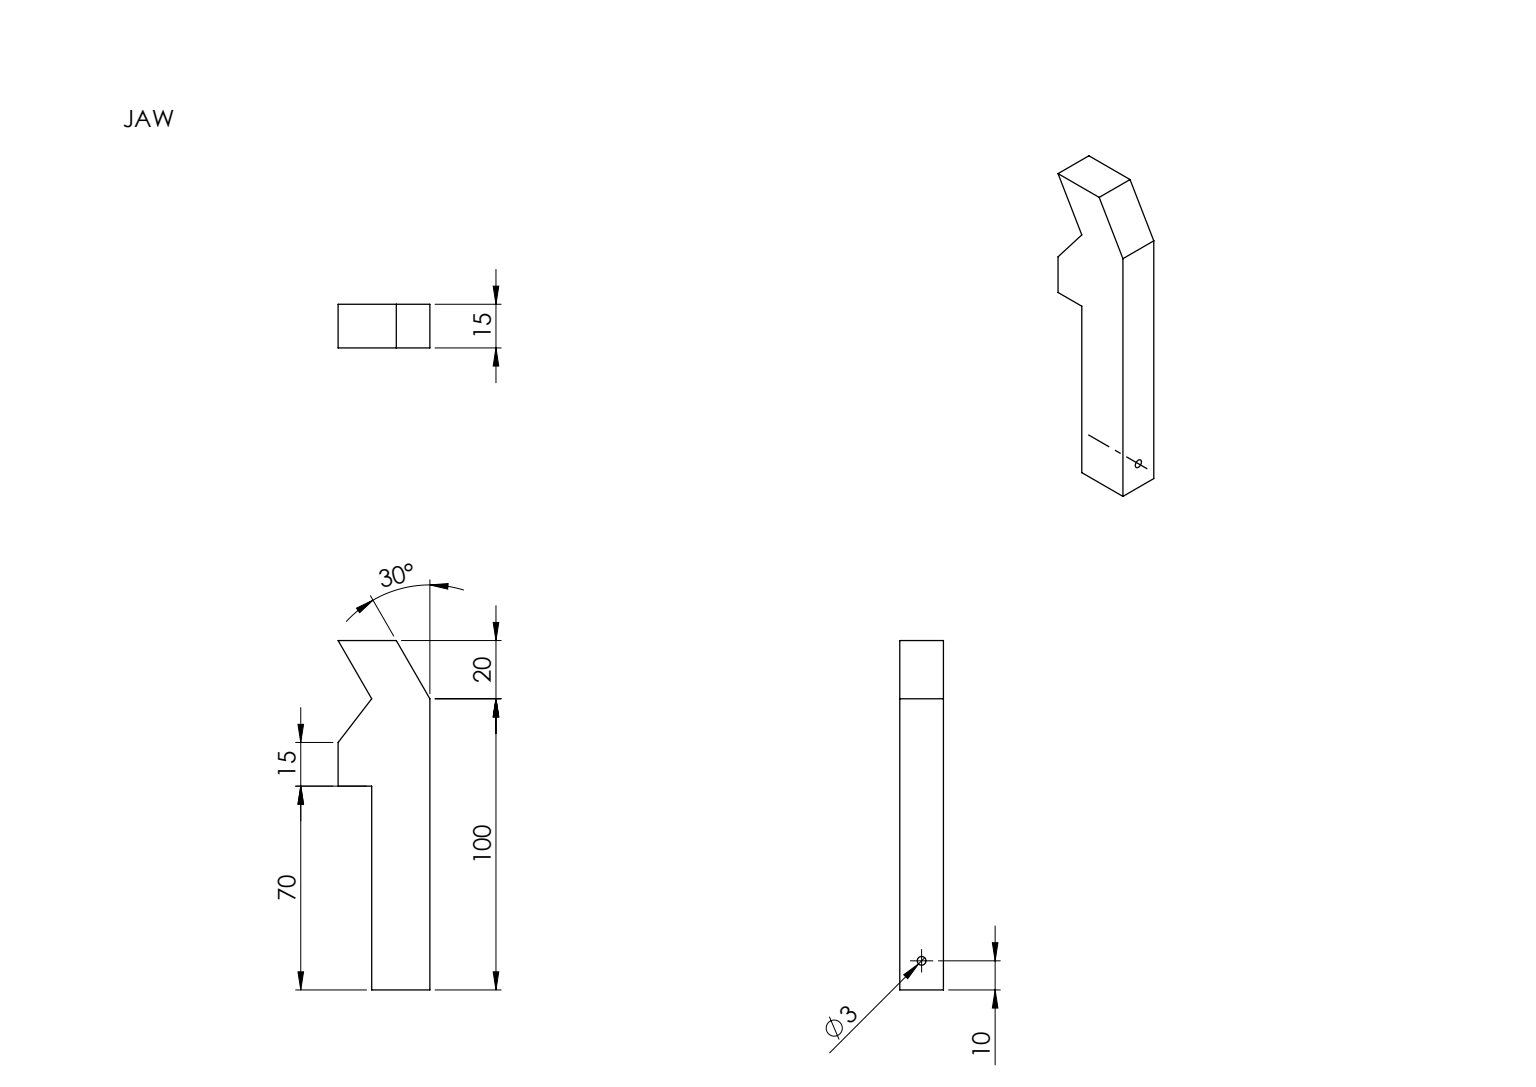
ISO-10303-21;
HEADER;
FILE_DESCRIPTION (('STEP AP214'),
    '1' );
FILE_NAME ('jaw.step',
    '2026-10-04T07:56:41',
    ( '' ),
    ( '' ),
    'SwSTEP 2.0',
    'SolidWorks 2026',
    '' );
FILE_SCHEMA (( 'AUTOMOTIVE_DESIGN' ));
ENDSEC;

DATA;
#13=SHAPE_DEFINITION_REPRESENTATION ( #5408, #1019 ) ;
#38=DIRECTION ( 'NONE',  ( -0.000000000000000000, -0.000000000000000000, -1.000000000000000000 ) ) ;
#42=VECTOR ( 'NONE', #3900, 1000.000000000000000 ) ;
#126=VECTOR ( 'NONE', #38, 1000.000000000000000 ) ;
#181=ORIENTED_EDGE ( 'NONE', *, *, #5142, .F. ) ;
#190=VECTOR ( 'NONE', #1369, 1000.000000000000000 ) ;
#227=ORIENTED_EDGE ( 'NONE', *, *, #6640, .F. ) ;
#250=VERTEX_POINT ( 'NONE', #3258 ) ;
#293=VERTEX_POINT ( 'NONE', #7045 ) ;
#304=ORIENTED_EDGE ( 'NONE', *, *, #4864, .F. ) ;
#353=EDGE_CURVE ( 'NONE', #6629, #3744, #7681, .T. ) ;
#393=CARTESIAN_POINT ( 'NONE',  ( 43.45299461620743386, -9.999999999999994671, 0.000000000000000000 ) ) ;
#417=VERTEX_POINT ( 'NONE', #8308 ) ;
#456=LINE ( 'NONE', #3663, #5763 ) ;
#466=PLANE ( 'NONE',  #7665 ) ;
#515=CIRCLE ( 'NONE', #4553, 1.500000000000000666 ) ;
#524=VERTEX_POINT ( 'NONE', #5948 ) ;
#534=VECTOR ( 'NONE', #7295, 1000.000000000000000 ) ;
#538=CARTESIAN_POINT ( 'NONE',  ( 43.45299461620744097, 100.0000000000000000, -7.500000000000000000 ) ) ;
#539=DIRECTION ( 'NONE',  ( -1.000000000000000000, 0.000000000000000000, 0.000000000000000000 ) ) ;
#549=VERTEX_POINT ( 'NONE', #4695 ) ;
#566=FACE_BOUND ( 'NONE', #6041, .T. ) ;
#573=CARTESIAN_POINT ( 'NONE',  ( 75.00000000000000000, -9.999999999999994671, 1.500000000000000666 ) ) ;
#576=EDGE_CURVE ( 'NONE', #1381, #2388, #1975, .T. ) ;
#579=CARTESIAN_POINT ( 'NONE',  ( 75.00000000000000000, -20.00000000000000000, -7.500000000000000000 ) ) ;
#605=CARTESIAN_POINT ( 'NONE',  ( 43.45299461620743386, 65.00000000000000000, 7.500000000000000000 ) ) ;
#617=ORIENTED_EDGE ( 'NONE', *, *, #2035, .T. ) ;
#635=ADVANCED_FACE ( 'NONE', ( #7236 ), #3406, .F. ) ;
#640=( NAMED_UNIT ( * ) PLANE_ANGLE_UNIT ( ) SI_UNIT ( $, .RADIAN. ) );
#646=VECTOR ( 'NONE', #7811, 1000.000000000000000 ) ;
#649=VECTOR ( 'NONE', #4755, 1000.000000000000000 ) ;
#653=CARTESIAN_POINT ( 'NONE',  ( 43.45299461620743386, 65.00000000000000000, 7.500000000000000000 ) ) ;
#701=ORIENTED_EDGE ( 'NONE', *, *, #4023, .T. ) ;
#712=APPLICATION_CONTEXT ( 'automotive_design' ) ;
#713=DIRECTION ( 'NONE',  ( -0.000000000000000000, -0.000000000000000000, -1.000000000000000000 ) ) ;
#714=LINE ( 'NONE', #5810, #3097 ) ;
#730=SURFACE_STYLE_USAGE ( .BOTH. , #5196 ) ;
#735=DIRECTION ( 'NONE',  ( -0.000000000000000000, 0.000000000000000000, -1.000000000000000000 ) ) ;
#746=ORIENTED_EDGE ( 'NONE', *, *, #4954, .T. ) ;
#773=EDGE_LOOP ( 'NONE', ( #701, #3537, #1533, #746 ) ) ;
#833=CARTESIAN_POINT ( 'NONE',  ( 54.99999999999999289, 80.00000000000000000, -7.500000000000000000 ) ) ;
#880=ORIENTED_EDGE ( 'NONE', *, *, #6640, .T. ) ;
#883=APPLICATION_CONTEXT ( 'automotive_design' ) ;
#896=UNCERTAINTY_MEASURE_WITH_UNIT (LENGTH_MEASURE( 1.000000000000000082E-05 ), #4515, 'distance_accuracy_value', 'NONE');
#906=PLANE ( 'NONE',  #6654 ) ;
#908=CARTESIAN_POINT ( 'NONE',  ( 75.00000000000000000, 80.00000000000000000, 7.500000000000000000 ) ) ;
#912=DIRECTION ( 'NONE',  ( 0.8660254037844380415, 0.5000000000000011102, -0.000000000000000000 ) ) ;
#939=ORIENTED_EDGE ( 'NONE', *, *, #6746, .T. ) ;
#940=CARTESIAN_POINT ( 'NONE',  ( 54.99999999999999289, 80.00000000000000000, -7.500000000000000000 ) ) ;
#949=MECHANICAL_DESIGN_GEOMETRIC_PRESENTATION_REPRESENTATION('',(#1216),#1896);
#955=SURFACE_SIDE_STYLE ('',( #6681 ) ) ;
#990=DIRECTION ( 'NONE',  ( 0.5000000000000011102, -0.8660254037844380415, 0.000000000000000000 ) ) ;
#997=CARTESIAN_POINT ( 'NONE',  ( 63.45299461620744808, 100.0000000000000000, 7.500000000000000000 ) ) ;
#999=ORIENTED_EDGE ( 'NONE', *, *, #7718, .T. ) ;
#1006=VECTOR ( 'NONE', #1758, 1000.000000000000114 ) ;
#1014=EDGE_LOOP ( 'NONE', ( #7055, #2724, #2403, #4042, #1733, #6191, #4300, #4661, #6588 ) ) ;
#1019=SHAPE_REPRESENTATION ( 'jaw', ( #2840 ), #1628 ) ;
#1038=DIRECTION ( 'NONE',  ( -0.000000000000000000, 0.000000000000000000, 1.000000000000000000 ) ) ;
#1049=MECHANICAL_DESIGN_GEOMETRIC_PRESENTATION_REPRESENTATION('',(#4809),#4356);
#1061=CARTESIAN_POINT ( 'NONE',  ( 75.00000000000000000, 80.00000000000000000, 7.500000000000000000 ) ) ;
#1080=ORIENTED_EDGE ( 'NONE', *, *, #5142, .T. ) ;
#1112=VECTOR ( 'NONE', #3807, 1000.000000000000000 ) ;
#1117=LINE ( 'NONE', #7526, #1006 ) ;
#1216=STYLED_ITEM ( 'NONE', ( #5735 ), #7608 ) ;
#1220=DIRECTION ( 'NONE',  ( 1.000000000000000000, -0.000000000000000000, -0.000000000000000000 ) ) ;
#1221=CARTESIAN_POINT ( 'NONE',  ( 75.00000000000000000, -20.00000000000000000, 7.500000000000000000 ) ) ;
#1242=CARTESIAN_POINT ( 'NONE',  ( 43.45299461620743386, -9.999999999999994671, 1.500000000000000666 ) ) ;
#1298=ORIENTED_EDGE ( 'NONE', *, *, #7183, .T. ) ;
#1326=DIRECTION ( 'NONE',  ( 1.000000000000000000, 0.000000000000000000, -0.000000000000000000 ) ) ;
#1369=DIRECTION ( 'NONE',  ( 1.000000000000000000, -0.000000000000000000, -0.000000000000000000 ) ) ;
#1381=VERTEX_POINT ( 'NONE', #5356 ) ;
#1447=ORIENTED_EDGE ( 'NONE', *, *, #5442, .T. ) ;
#1468=AXIS2_PLACEMENT_3D ( 'NONE', #3072, #1220, #4965 ) ;
#1533=ORIENTED_EDGE ( 'NONE', *, *, #7718, .F. ) ;
#1537=FACE_OUTER_BOUND ( 'NONE', #1693, .T. ) ;
#1546=( NAMED_UNIT ( * ) PLANE_ANGLE_UNIT ( ) SI_UNIT ( $, .RADIAN. ) );
#1548=EDGE_CURVE ( 'NONE', #5519, #1381, #5167, .T. ) ;
#1591=DIRECTION ( 'NONE',  ( -0.6099942813304201072, -0.7924058156930603447, 0.000000000000000000 ) ) ;
#1623=VECTOR ( 'NONE', #1650, 1000.000000000000000 ) ;
#1628=( GEOMETRIC_REPRESENTATION_CONTEXT ( 3 ) GLOBAL_UNCERTAINTY_ASSIGNED_CONTEXT ( ( #4856 ) ) GLOBAL_UNIT_ASSIGNED_CONTEXT ( ( #2005, #6383, #3771 ) ) REPRESENTATION_CONTEXT ( 'NONE', 'WORKASPACE' ) );
#1649=VERTEX_POINT ( 'NONE', #573 ) ;
#1650=DIRECTION ( 'NONE',  ( -1.000000000000000000, 0.000000000000000000, 0.000000000000000000 ) ) ;
#1659=EDGE_CURVE ( 'NONE', #250, #417, #4402, .T. ) ;
#1667=CARTESIAN_POINT ( 'NONE',  ( 43.45299461620744097, 100.0000000000000000, -7.500000000000000000 ) ) ;
#1676=VECTOR ( 'NONE', #7231, 1000.000000000000000 ) ;
#1690=MANIFOLD_SOLID_BREP ( 'Cut-Extrude1', #5315 ) ;
#1691=ORIENTED_EDGE ( 'NONE', *, *, #2448, .T. ) ;
#1693=EDGE_LOOP ( 'NONE', ( #2245, #2702, #999, #617, #3311, #7489, #1691, #2350, #6749 ) ) ;
#1721=ADVANCED_FACE ( 'NONE', ( #4785 ), #5294, .F. ) ;
#1725=EDGE_CURVE ( 'NONE', #1381, #6629, #3483, .T. ) ;
#1733=ORIENTED_EDGE ( 'NONE', *, *, #2960, .F. ) ;
#1756=DIRECTION ( 'NONE',  ( 1.000000000000000000, 0.000000000000000000, 0.000000000000000000 ) ) ;
#1758=DIRECTION ( 'NONE',  ( -0.5000000000000011102, 0.8660254037844380415, 0.000000000000000000 ) ) ;
#1781=EDGE_CURVE ( 'NONE', #293, #5112, #4033, .T. ) ;
#1792=LINE ( 'NONE', #5025, #4464 ) ;
#1841=VERTEX_POINT ( 'NONE', #997 ) ;
#1842=LINE ( 'NONE', #7145, #3688 ) ;
#1856=ORIENTED_EDGE ( 'NONE', *, *, #1548, .F. ) ;
#1885=CARTESIAN_POINT ( 'NONE',  ( 54.99999999999999289, 50.00000000000000000, 7.500000000000000000 ) ) ;
#1895=DIRECTION ( 'NONE',  ( 1.000000000000000000, 0.000000000000000000, 0.000000000000000000 ) ) ;
#1896=( GEOMETRIC_REPRESENTATION_CONTEXT ( 3 ) GLOBAL_UNCERTAINTY_ASSIGNED_CONTEXT ( ( #896 ) ) GLOBAL_UNIT_ASSIGNED_CONTEXT ( ( #4515, #640, #7095 ) ) REPRESENTATION_CONTEXT ( 'NONE', 'WORKASPACE' ) );
#1899=ORIENTED_EDGE ( 'NONE', *, *, #4820, .F. ) ;
#1913=ADVANCED_FACE ( 'NONE', ( #4275 ), #2936, .F. ) ;
#1922=VERTEX_POINT ( 'NONE', #3564 ) ;
#1943=ORIENTED_EDGE ( 'NONE', *, *, #2448, .F. ) ;
#1975=LINE ( 'NONE', #7195, #7322 ) ;
#2005=( LENGTH_UNIT ( ) NAMED_UNIT ( * ) SI_UNIT ( .MILLI., .METRE. ) );
#2017=PRODUCT_DEFINITION ( 'UNKNOWN', '', #4690, #4178 ) ;
#2035=EDGE_CURVE ( 'NONE', #8322, #1841, #1117, .T. ) ;
#2076=DIRECTION ( 'NONE',  ( 0.5000000000000011102, -0.8660254037844380415, 0.000000000000000000 ) ) ;
#2097=DIRECTION ( 'NONE',  ( 0.000000000000000000, 0.000000000000000000, -1.000000000000000000 ) ) ;
#2148=ORIENTED_EDGE ( 'NONE', *, *, #3348, .F. ) ;
#2170=EDGE_LOOP ( 'NONE', ( #5540, #6001, #8319, #4192 ) ) ;
#2178=EDGE_CURVE ( 'NONE', #5519, #3650, #1842, .T. ) ;
#2200=EDGE_LOOP ( 'NONE', ( #1298, #7014, #1856, #8055 ) ) ;
#2213=ORIENTED_EDGE ( 'NONE', *, *, #3070, .T. ) ;
#2221=LINE ( 'NONE', #7269, #6382 ) ;
#2245=ORIENTED_EDGE ( 'NONE', *, *, #2667, .T. ) ;
#2271=CARTESIAN_POINT ( 'NONE',  ( 75.00000000000000000, -20.00000000000000000, 7.500000000000000000 ) ) ;
#2323=ORIENTED_EDGE ( 'NONE', *, *, #2035, .F. ) ;
#2334=EDGE_LOOP ( 'NONE', ( #181, #6990 ) ) ;
#2348=VECTOR ( 'NONE', #5444, 1000.000000000000000 ) ;
#2350=ORIENTED_EDGE ( 'NONE', *, *, #1548, .T. ) ;
#2373=LINE ( 'NONE', #4175, #2348 ) ;
#2388=VERTEX_POINT ( 'NONE', #1885 ) ;
#2393=EDGE_CURVE ( 'NONE', #5386, #1649, #4518, .T. ) ;
#2403=ORIENTED_EDGE ( 'NONE', *, *, #7183, .F. ) ;
#2412=CARTESIAN_POINT ( 'NONE',  ( 54.99999999999999289, -20.00000000000000000, 7.500000000000000000 ) ) ;
#2445=ORIENTED_EDGE ( 'NONE', *, *, #7652, .T. ) ;
#2448=EDGE_CURVE ( 'NONE', #524, #5519, #8279, .T. ) ;
#2453=FACE_OUTER_BOUND ( 'NONE', #3610, .T. ) ;
#2455=CARTESIAN_POINT ( 'NONE',  ( 43.45299461620743386, 65.00000000000000000, -7.500000000000000000 ) ) ;
#2467=ORIENTED_EDGE ( 'NONE', *, *, #7477, .T. ) ;
#2471=ORIENTED_EDGE ( 'NONE', *, *, #6088, .T. ) ;
#2488=CARTESIAN_POINT ( 'NONE',  ( 54.99999999999999289, -20.00000000000000000, 7.500000000000000000 ) ) ;
#2507=FILL_AREA_STYLE ('',( #7013 ) ) ;
#2525=PRODUCT ( 'jaw', 'jaw', '', ( #5784 ) ) ;
#2535=DIRECTION ( 'NONE',  ( -0.8660254037844380415, -0.5000000000000011102, 0.000000000000000000 ) ) ;
#2551=CARTESIAN_POINT ( 'NONE',  ( 54.99999999999999289, 80.00000000000000000, 7.500000000000000000 ) ) ;
#2585=CARTESIAN_POINT ( 'NONE',  ( 63.45299461620744808, 100.0000000000000000, 7.500000000000000000 ) ) ;
#2637=EDGE_CURVE ( 'NONE', #1922, #549, #4649, .T. ) ;
#2667=EDGE_CURVE ( 'NONE', #2388, #4058, #2221, .T. ) ;
#2676=CARTESIAN_POINT ( 'NONE',  ( 43.45299461620743386, 65.00000000000000000, -7.500000000000000000 ) ) ;
#2685=CARTESIAN_POINT ( 'NONE',  ( 54.99999999999999289, -9.999999999999994671, 0.000000000000000000 ) ) ;
#2702=ORIENTED_EDGE ( 'NONE', *, *, #4820, .T. ) ;
#2724=ORIENTED_EDGE ( 'NONE', *, *, #353, .F. ) ;
#2760=ADVANCED_FACE ( 'NONE', ( #1537 ), #906, .T. ) ;
#2783=EDGE_LOOP ( 'NONE', ( #227, #3912, #3895, #4312 ) ) ;
#2801=ORIENTED_EDGE ( 'NONE', *, *, #576, .F. ) ;
#2805=VECTOR ( 'NONE', #3237, 1000.000000000000000 ) ;
#2818=CARTESIAN_POINT ( 'NONE',  ( 63.45299461620744808, 100.0000000000000000, 7.500000000000000000 ) ) ;
#2840=AXIS2_PLACEMENT_3D ( 'NONE', #8120, #5497, #1756 ) ;
#2850=CARTESIAN_POINT ( 'NONE',  ( 0.000000000000000000, 0.000000000000000000, 7.500000000000000000 ) ) ;
#2856=ADVANCED_FACE ( 'NONE', ( #4986 ), #5457, .F. ) ;
#2871=CARTESIAN_POINT ( 'NONE',  ( 75.00000000000000000, -9.999999999999994671, 0.000000000000000000 ) ) ;
#2888=VECTOR ( 'NONE', #7689, 1000.000000000000114 ) ;
#2923=DIRECTION ( 'NONE',  ( 1.000000000000000000, 0.000000000000000000, 0.000000000000000000 ) ) ;
#2936=PLANE ( 'NONE',  #3559 ) ;
#2960=EDGE_CURVE ( 'NONE', #5449, #6860, #4819, .T. ) ;
#3015=VECTOR ( 'NONE', #7593, 1000.000000000000000 ) ;
#3016=UNCERTAINTY_MEASURE_WITH_UNIT (LENGTH_MEASURE( 1.000000000000000082E-05 ), #7238, 'distance_accuracy_value', 'NONE');
#3070=EDGE_CURVE ( 'NONE', #8322, #293, #5574, .T. ) ;
#3072=CARTESIAN_POINT ( 'NONE',  ( 43.45299461620743386, -9.999999999999994671, 0.000000000000000000 ) ) ;
#3097=VECTOR ( 'NONE', #6576, 1000.000000000000000 ) ;
#3126=EDGE_LOOP ( 'NONE', ( #5435, #6018, #2801, #7528 ) ) ;
#3144=CARTESIAN_POINT ( 'NONE',  ( 54.99999999999999289, 50.00000000000000000, 7.500000000000000000 ) ) ;
#3146=AXIS2_PLACEMENT_3D ( 'NONE', #6708, #7871, #2097 ) ;
#3214=EDGE_CURVE ( 'NONE', #1841, #4787, #5653, .T. ) ;
#3237=DIRECTION ( 'NONE',  ( 9.251858538542971828E-16, -1.000000000000000000, 0.000000000000000000 ) ) ;
#3254=CARTESIAN_POINT ( 'NONE',  ( 43.45299461620744808, 50.00000000000000000, 7.500000000000000000 ) ) ;
#3258=CARTESIAN_POINT ( 'NONE',  ( 54.99999999999999289, -20.00000000000000000, -7.500000000000000000 ) ) ;
#3311=ORIENTED_EDGE ( 'NONE', *, *, #3214, .T. ) ;
#3338=DIRECTION ( 'NONE',  ( 0.000000000000000000, 1.000000000000000000, 0.000000000000000000 ) ) ;
#3348=EDGE_CURVE ( 'NONE', #4787, #524, #1792, .T. ) ;
#3406=PLANE ( 'NONE',  #5741 ) ;
#3423=CARTESIAN_POINT ( 'NONE',  ( 63.45299461620744808, 100.0000000000000000, -7.500000000000000000 ) ) ;
#3462=CARTESIAN_POINT ( 'NONE',  ( 75.00000000000000000, -20.00000000000000000, 7.500000000000000000 ) ) ;
#3482=ORIENTED_EDGE ( 'NONE', *, *, #5442, .F. ) ;
#3483=LINE ( 'NONE', #7197, #5034 ) ;
#3487=DIRECTION ( 'NONE',  ( 0.000000000000000000, -1.000000000000000000, 0.000000000000000000 ) ) ;
#3537=ORIENTED_EDGE ( 'NONE', *, *, #3070, .F. ) ;
#3559=AXIS2_PLACEMENT_3D ( 'NONE', #4949, #1038, #4874 ) ;
#3564=CARTESIAN_POINT ( 'NONE',  ( 54.99999999999999289, -9.999999999999994671, -1.500000000000000666 ) ) ;
#3610=EDGE_LOOP ( 'NONE', ( #7750, #5914, #1899, #939 ) ) ;
#3623=FACE_OUTER_BOUND ( 'NONE', #4276, .T. ) ;
#3650=VERTEX_POINT ( 'NONE', #2676 ) ;
#3663=CARTESIAN_POINT ( 'NONE',  ( 63.45299461620744808, 100.0000000000000000, 7.500000000000000000 ) ) ;
#3675=LINE ( 'NONE', #2455, #3015 ) ;
#3685=CIRCLE ( 'NONE', #4615, 1.500000000000000666 ) ;
#3688=VECTOR ( 'NONE', #5113, 1000.000000000000000 ) ;
#3716=DIRECTION ( 'NONE',  ( 0.000000000000000000, -0.000000000000000000, 1.000000000000000000 ) ) ;
#3744=VERTEX_POINT ( 'NONE', #6155 ) ;
#3745=DIRECTION ( 'NONE',  ( -0.000000000000000000, -0.000000000000000000, -1.000000000000000000 ) ) ;
#3746=PLANE ( 'NONE',  #5432 ) ;
#3771=( NAMED_UNIT ( * ) SI_UNIT ( $, .STERADIAN. ) SOLID_ANGLE_UNIT ( ) );
#3807=DIRECTION ( 'NONE',  ( -1.000000000000000000, 0.000000000000000000, 0.000000000000000000 ) ) ;
#3815=VECTOR ( 'NONE', #5130, 1000.000000000000000 ) ;
#3852=EDGE_CURVE ( 'NONE', #3744, #250, #2373, .T. ) ;
#3872=ORIENTED_EDGE ( 'NONE', *, *, #7477, .F. ) ;
#3892=AXIS2_PLACEMENT_3D ( 'NONE', #2818, #3487, #7243 ) ;
#3895=ORIENTED_EDGE ( 'NONE', *, *, #6954, .T. ) ;
#3900=DIRECTION ( 'NONE',  ( -0.000000000000000000, -0.000000000000000000, -1.000000000000000000 ) ) ;
#3912=ORIENTED_EDGE ( 'NONE', *, *, #2393, .T. ) ;
#3938=DIRECTION ( 'NONE',  ( 1.000000000000000000, 0.000000000000000000, 0.000000000000000000 ) ) ;
#3944=CARTESIAN_POINT ( 'NONE',  ( 54.99999999999999289, 80.00000000000000000, 7.500000000000000000 ) ) ;
#3965=VECTOR ( 'NONE', #5376, 1000.000000000000114 ) ;
#3966=CARTESIAN_POINT ( 'NONE',  ( 54.99999999999999289, 80.00000000000000000, 7.500000000000000000 ) ) ;
#4006=CARTESIAN_POINT ( 'NONE',  ( 54.99999999999999289, -20.00000000000000000, 7.500000000000000000 ) ) ;
#4023=EDGE_CURVE ( 'NONE', #417, #293, #6401, .T. ) ;
#4032=DIRECTION ( 'NONE',  ( 1.000000000000000000, 0.000000000000000000, 0.000000000000000000 ) ) ;
#4033=LINE ( 'NONE', #5927, #3965 ) ;
#4042=ORIENTED_EDGE ( 'NONE', *, *, #6088, .F. ) ;
#4058=VERTEX_POINT ( 'NONE', #2488 ) ;
#4108=ADVANCED_FACE ( 'NONE', ( #5006, #6277 ), #3746, .F. ) ;
#4112=EDGE_LOOP ( 'NONE', ( #5128, #304, #2148, #2467 ) ) ;
#4136=VECTOR ( 'NONE', #1895, 1000.000000000000000 ) ;
#4155=AXIS2_PLACEMENT_3D ( 'NONE', #1061, #2535, #2076 ) ;
#4175=CARTESIAN_POINT ( 'NONE',  ( 54.99999999999999289, 50.00000000000000000, -7.500000000000000000 ) ) ;
#4178=PRODUCT_DEFINITION_CONTEXT ( 'detailed design', #712, 'design' ) ;
#4180=CARTESIAN_POINT ( 'NONE',  ( 75.00000000000000000, -9.999999999999994671, 0.000000000000000000 ) ) ;
#4192=ORIENTED_EDGE ( 'NONE', *, *, #4808, .T. ) ;
#4257=PLANE ( 'NONE',  #4155 ) ;
#4275=FACE_OUTER_BOUND ( 'NONE', #1014, .T. ) ;
#4276=EDGE_LOOP ( 'NONE', ( #8174, #6317, #4791, #1080 ) ) ;
#4300=ORIENTED_EDGE ( 'NONE', *, *, #1781, .F. ) ;
#4312=ORIENTED_EDGE ( 'NONE', *, *, #2637, .F. ) ;
#4356=( GEOMETRIC_REPRESENTATION_CONTEXT ( 3 ) GLOBAL_UNCERTAINTY_ASSIGNED_CONTEXT ( ( #3016 ) ) GLOBAL_UNIT_ASSIGNED_CONTEXT ( ( #7238, #1546, #7917 ) ) REPRESENTATION_CONTEXT ( 'NONE', 'WORKASPACE' ) );
#4395=PLANE ( 'NONE',  #7317 ) ;
#4402=LINE ( 'NONE', #6981, #4136 ) ;
#4419=VECTOR ( 'NONE', #713, 1000.000000000000000 ) ;
#4438=PLANE ( 'NONE',  #5968 ) ;
#4464=VECTOR ( 'NONE', #5690, 1000.000000000000114 ) ;
#4499=ADVANCED_FACE ( 'NONE', ( #2453 ), #466, .F. ) ;
#4515=( LENGTH_UNIT ( ) NAMED_UNIT ( * ) SI_UNIT ( .MILLI., .METRE. ) );
#4518=LINE ( 'NONE', #1242, #190 ) ;
#4520=LINE ( 'NONE', #7101, #42 ) ;
#4526=DIRECTION ( 'NONE',  ( 0.6099942813304201072, 0.7924058156930603447, 0.000000000000000000 ) ) ;
#4544=LINE ( 'NONE', #3966, #4419 ) ;
#4553=AXIS2_PLACEMENT_3D ( 'NONE', #2871, #5350, #6780 ) ;
#4567=DIRECTION ( 'NONE',  ( 0.7924058156930603447, -0.6099942813304201072, 0.000000000000000000 ) ) ;
#4615=AXIS2_PLACEMENT_3D ( 'NONE', #2685, #1326, #8323 ) ;
#4643=ORIENTED_EDGE ( 'NONE', *, *, #6814, .T. ) ;
#4649=LINE ( 'NONE', #4687, #1676 ) ;
#4660=ADVANCED_FACE ( 'NONE', ( #8303 ), #4257, .F. ) ;
#4661=ORIENTED_EDGE ( 'NONE', *, *, #4023, .F. ) ;
#4687=CARTESIAN_POINT ( 'NONE',  ( 43.45299461620743386, -9.999999999999994671, -1.500000000000000666 ) ) ;
#4690=PRODUCT_DEFINITION_FORMATION_WITH_SPECIFIED_SOURCE ( 'ANY', '', #2525, .NOT_KNOWN. ) ;
#4695=CARTESIAN_POINT ( 'NONE',  ( 75.00000000000000000, -9.999999999999994671, -1.500000000000000666 ) ) ;
#4697=FILL_AREA_STYLE ('',( #6724 ) ) ;
#4738=SURFACE_STYLE_USAGE ( .BOTH. , #955 ) ;
#4755=DIRECTION ( 'NONE',  ( -0.000000000000000000, -0.000000000000000000, -1.000000000000000000 ) ) ;
#4785=FACE_OUTER_BOUND ( 'NONE', #4112, .T. ) ;
#4786=ADVANCED_FACE ( 'NONE', ( #7806 ), #6491, .F. ) ;
#4787=VERTEX_POINT ( 'NONE', #5767 ) ;
#4791=ORIENTED_EDGE ( 'NONE', *, *, #2637, .T. ) ;
#4808=EDGE_CURVE ( 'NONE', #2388, #3744, #7169, .T. ) ;
#4809=STYLED_ITEM ( 'NONE', ( #7277 ), #1690 ) ;
#4819=LINE ( 'NONE', #1667, #6108 ) ;
#4820=EDGE_CURVE ( 'NONE', #4058, #6070, #5138, .T. ) ;
#4831=VECTOR ( 'NONE', #5098, 1000.000000000000000 ) ;
#4856=UNCERTAINTY_MEASURE_WITH_UNIT (LENGTH_MEASURE( 1.000000000000000082E-05 ), #2005, 'distance_accuracy_value', 'NONE');
#4864=EDGE_CURVE ( 'NONE', #524, #6860, #4544, .T. ) ;
#4874=DIRECTION ( 'NONE',  ( 1.000000000000000000, 0.000000000000000000, 0.000000000000000000 ) ) ;
#4945=CARTESIAN_POINT ( 'NONE',  ( 75.00000000000000000, 80.00000000000000000, 7.500000000000000000 ) ) ;
#4949=CARTESIAN_POINT ( 'NONE',  ( 0.000000000000000000, 0.000000000000000000, -7.500000000000000000 ) ) ;
#4954=EDGE_CURVE ( 'NONE', #6070, #417, #6069, .T. ) ;
#4965=DIRECTION ( 'NONE',  ( 0.000000000000000000, 0.000000000000000000, -1.000000000000000000 ) ) ;
#4986=FACE_OUTER_BOUND ( 'NONE', #2783, .T. ) ;
#5006=FACE_BOUND ( 'NONE', #2334, .T. ) ;
#5025=CARTESIAN_POINT ( 'NONE',  ( 43.45299461620744097, 100.0000000000000000, 7.500000000000000000 ) ) ;
#5034=VECTOR ( 'NONE', #6010, 1000.000000000000000 ) ;
#5048=CARTESIAN_POINT ( 'NONE',  ( 54.99999999999999289, -9.999999999999994671, 1.500000000000000666 ) ) ;
#5069=SHAPE_REPRESENTATION_RELATIONSHIP ( 'NONE' , 'NONE' ,  #1019, #7608 ) ;
#5098=DIRECTION ( 'NONE',  ( 1.000000000000000000, 0.000000000000000000, 0.000000000000000000 ) ) ;
#5112=VERTEX_POINT ( 'NONE', #3423 ) ;
#5113=DIRECTION ( 'NONE',  ( -0.000000000000000000, -0.000000000000000000, -1.000000000000000000 ) ) ;
#5117=CARTESIAN_POINT ( 'NONE',  ( 43.45299461620744808, 50.00000000000000000, -7.500000000000000000 ) ) ;
#5128=ORIENTED_EDGE ( 'NONE', *, *, #2960, .T. ) ;
#5130=DIRECTION ( 'NONE',  ( 0.000000000000000000, 1.000000000000000000, 0.000000000000000000 ) ) ;
#5138=LINE ( 'NONE', #4006, #4831 ) ;
#5142=EDGE_CURVE ( 'NONE', #549, #1649, #515, .T. ) ;
#5159=AXIS2_PLACEMENT_3D ( 'NONE', #4180, #2923, #6202 ) ;
#5167=LINE ( 'NONE', #653, #2805 ) ;
#5196=SURFACE_SIDE_STYLE ('',( #6968 ) ) ;
#5251=CARTESIAN_POINT ( 'NONE',  ( 43.45299461620744097, 100.0000000000000000, 7.500000000000000000 ) ) ;
#5294=PLANE ( 'NONE',  #7881 ) ;
#5315=CLOSED_SHELL ( 'NONE', ( #2856, #6616, #4499, #4108, #4660, #5872, #1721, #635, #6612, #4786, #2760, #1913, #5347 ) ) ;
#5347=ADVANCED_FACE ( 'NONE', ( #3623 ), #7501, .F. ) ;
#5350=DIRECTION ( 'NONE',  ( 1.000000000000000000, 0.000000000000000000, 0.000000000000000000 ) ) ;
#5352=CARTESIAN_POINT ( 'NONE',  ( 63.45299461620744808, 100.0000000000000000, -7.500000000000000000 ) ) ;
#5356=CARTESIAN_POINT ( 'NONE',  ( 43.45299461620744808, 50.00000000000000000, 7.500000000000000000 ) ) ;
#5376=DIRECTION ( 'NONE',  ( -0.5000000000000011102, 0.8660254037844380415, 0.000000000000000000 ) ) ;
#5386=VERTEX_POINT ( 'NONE', #5048 ) ;
#5408=PRODUCT_DEFINITION_SHAPE ( 'NONE', 'NONE',  #2017 ) ;
#5422=LINE ( 'NONE', #833, #7450 ) ;
#5432=AXIS2_PLACEMENT_3D ( 'NONE', #1221, #539, #7668 ) ;
#5435=ORIENTED_EDGE ( 'NONE', *, *, #353, .T. ) ;
#5442=EDGE_CURVE ( 'NONE', #1841, #5112, #456, .T. ) ;
#5444=DIRECTION ( 'NONE',  ( 0.000000000000000000, -1.000000000000000000, 0.000000000000000000 ) ) ;
#5449=VERTEX_POINT ( 'NONE', #538 ) ;
#5457=CYLINDRICAL_SURFACE ( 'NONE', #8000, 1.500000000000000666 ) ;
#5497=DIRECTION ( 'NONE',  ( 0.000000000000000000, 0.000000000000000000, 1.000000000000000000 ) ) ;
#5518=CARTESIAN_POINT ( 'NONE',  ( 43.45299461620743386, 65.00000000000000000, 7.500000000000000000 ) ) ;
#5519=VERTEX_POINT ( 'NONE', #5518 ) ;
#5540=ORIENTED_EDGE ( 'NONE', *, *, #3852, .T. ) ;
#5574=LINE ( 'NONE', #4945, #7189 ) ;
#5592=EDGE_LOOP ( 'NONE', ( #2471, #8176, #1943, #7923 ) ) ;
#5653=LINE ( 'NONE', #2585, #1112 ) ;
#5690=DIRECTION ( 'NONE',  ( 0.5000000000000011102, -0.8660254037844380415, 0.000000000000000000 ) ) ;
#5735=PRESENTATION_STYLE_ASSIGNMENT (( #730 ) ) ;
#5741=AXIS2_PLACEMENT_3D ( 'NONE', #3944, #4567, #4526 ) ;
#5742=FACE_OUTER_BOUND ( 'NONE', #2170, .T. ) ;
#5755=FACE_OUTER_BOUND ( 'NONE', #7669, .T. ) ;
#5763=VECTOR ( 'NONE', #3745, 1000.000000000000000 ) ;
#5767=CARTESIAN_POINT ( 'NONE',  ( 43.45299461620744097, 100.0000000000000000, 7.500000000000000000 ) ) ;
#5784=PRODUCT_CONTEXT ( 'NONE', #883, 'mechanical' ) ;
#5809=CARTESIAN_POINT ( 'NONE',  ( 54.99999999999999289, 50.00000000000000000, 7.500000000000000000 ) ) ;
#5810=CARTESIAN_POINT ( 'NONE',  ( 43.45299461620744097, 100.0000000000000000, 7.500000000000000000 ) ) ;
#5826=CIRCLE ( 'NONE', #3146, 1.500000000000000666 ) ;
#5872=ADVANCED_FACE ( 'NONE', ( #5755 ), #7944, .F. ) ;
#5884=COLOUR_RGB ( '', 0.09019608, 0.27058824, 0.51372549) ;
#5914=ORIENTED_EDGE ( 'NONE', *, *, #4954, .F. ) ;
#5927=CARTESIAN_POINT ( 'NONE',  ( 75.00000000000000000, 80.00000000000000000, -7.500000000000000000 ) ) ;
#5948=CARTESIAN_POINT ( 'NONE',  ( 54.99999999999999289, 80.00000000000000000, 7.500000000000000000 ) ) ;
#5968=AXIS2_PLACEMENT_3D ( 'NONE', #605, #6426, #6511 ) ;
#5970=DIRECTION ( 'NONE',  ( -0.5000000000000011102, 0.8660254037844380415, 0.000000000000000000 ) ) ;
#6001=ORIENTED_EDGE ( 'NONE', *, *, #6746, .F. ) ;
#6010=DIRECTION ( 'NONE',  ( -0.000000000000000000, -0.000000000000000000, -1.000000000000000000 ) ) ;
#6018=ORIENTED_EDGE ( 'NONE', *, *, #4808, .F. ) ;
#6041=EDGE_LOOP ( 'NONE', ( #4643, #880 ) ) ;
#6069=LINE ( 'NONE', #3462, #649 ) ;
#6070=VERTEX_POINT ( 'NONE', #2271 ) ;
#6087=DIRECTION ( 'NONE',  ( 1.000000000000000000, -0.000000000000000000, -0.000000000000000000 ) ) ;
#6088=EDGE_CURVE ( 'NONE', #6860, #3650, #5422, .T. ) ;
#6091=EDGE_LOOP ( 'NONE', ( #6160, #3482, #2323, #2213 ) ) ;
#6108=VECTOR ( 'NONE', #990, 1000.000000000000114 ) ;
#6155=CARTESIAN_POINT ( 'NONE',  ( 54.99999999999999289, 50.00000000000000000, -7.500000000000000000 ) ) ;
#6160=ORIENTED_EDGE ( 'NONE', *, *, #1781, .T. ) ;
#6191=ORIENTED_EDGE ( 'NONE', *, *, #7652, .F. ) ;
#6202=DIRECTION ( 'NONE',  ( 0.000000000000000000, 0.000000000000000000, -1.000000000000000000 ) ) ;
#6277=FACE_OUTER_BOUND ( 'NONE', #773, .T. ) ;
#6286=DIRECTION ( 'NONE',  ( 0.000000000000000000, 1.000000000000000000, 0.000000000000000000 ) ) ;
#6317=ORIENTED_EDGE ( 'NONE', *, *, #6814, .F. ) ;
#6382=VECTOR ( 'NONE', #6631, 1000.000000000000000 ) ;
#6383=( NAMED_UNIT ( * ) PLANE_ANGLE_UNIT ( ) SI_UNIT ( $, .RADIAN. ) );
#6388=FACE_OUTER_BOUND ( 'NONE', #2200, .T. ) ;
#6401=LINE ( 'NONE', #579, #3815 ) ;
#6426=DIRECTION ( 'NONE',  ( 1.000000000000000000, 9.251858538542971828E-16, -0.000000000000000000 ) ) ;
#6491=PLANE ( 'NONE',  #7400 ) ;
#6511=DIRECTION ( 'NONE',  ( -9.251858538542971828E-16, 1.000000000000000000, 0.000000000000000000 ) ) ;
#6576=DIRECTION ( 'NONE',  ( -0.000000000000000000, -0.000000000000000000, -1.000000000000000000 ) ) ;
#6588=ORIENTED_EDGE ( 'NONE', *, *, #1659, .F. ) ;
#6612=ADVANCED_FACE ( 'NONE', ( #6388 ), #4438, .F. ) ;
#6616=ADVANCED_FACE ( 'NONE', ( #566, #5742 ), #4395, .F. ) ;
#6629=VERTEX_POINT ( 'NONE', #5117 ) ;
#6631=DIRECTION ( 'NONE',  ( 0.000000000000000000, -1.000000000000000000, 0.000000000000000000 ) ) ;
#6640=EDGE_CURVE ( 'NONE', #5386, #1922, #3685, .T. ) ;
#6654=AXIS2_PLACEMENT_3D ( 'NONE', #2850, #7991, #3938 ) ;
#6681=SURFACE_STYLE_FILL_AREA ( #4697 ) ;
#6708=CARTESIAN_POINT ( 'NONE',  ( 54.99999999999999289, -9.999999999999994671, 0.000000000000000000 ) ) ;
#6717=DIRECTION ( 'NONE',  ( 0.000000000000000000, 0.000000000000000000, -1.000000000000000000 ) ) ;
#6724=FILL_AREA_STYLE_COLOUR ( '', #5884 ) ;
#6746=EDGE_CURVE ( 'NONE', #4058, #250, #4520, .T. ) ;
#6749=ORIENTED_EDGE ( 'NONE', *, *, #576, .T. ) ;
#6780=DIRECTION ( 'NONE',  ( 0.000000000000000000, 0.000000000000000000, -1.000000000000000000 ) ) ;
#6814=EDGE_CURVE ( 'NONE', #1922, #5386, #5826, .T. ) ;
#6860=VERTEX_POINT ( 'NONE', #940 ) ;
#6954=EDGE_CURVE ( 'NONE', #1649, #549, #7051, .T. ) ;
#6968=SURFACE_STYLE_FILL_AREA ( #2507 ) ;
#6981=CARTESIAN_POINT ( 'NONE',  ( 54.99999999999999289, -20.00000000000000000, -7.500000000000000000 ) ) ;
#6990=ORIENTED_EDGE ( 'NONE', *, *, #6954, .F. ) ;
#7013=FILL_AREA_STYLE_COLOUR ( '', #8216 ) ;
#7014=ORIENTED_EDGE ( 'NONE', *, *, #1725, .F. ) ;
#7018=DIRECTION ( 'NONE',  ( 1.000000000000000000, 0.000000000000000000, -0.000000000000000000 ) ) ;
#7040=DIRECTION ( 'NONE',  ( 0.000000000000000000, -0.000000000000000000, 1.000000000000000000 ) ) ;
#7045=CARTESIAN_POINT ( 'NONE',  ( 75.00000000000000000, 80.00000000000000000, -7.500000000000000000 ) ) ;
#7051=CIRCLE ( 'NONE', #5159, 1.500000000000000666 ) ;
#7055=ORIENTED_EDGE ( 'NONE', *, *, #3852, .F. ) ;
#7095=( NAMED_UNIT ( * ) SI_UNIT ( $, .STERADIAN. ) SOLID_ANGLE_UNIT ( ) );
#7101=CARTESIAN_POINT ( 'NONE',  ( 54.99999999999999289, -20.00000000000000000, 7.500000000000000000 ) ) ;
#7145=CARTESIAN_POINT ( 'NONE',  ( 43.45299461620743386, 65.00000000000000000, 7.500000000000000000 ) ) ;
#7169=LINE ( 'NONE', #5809, #126 ) ;
#7183=EDGE_CURVE ( 'NONE', #3650, #6629, #3675, .T. ) ;
#7189=VECTOR ( 'NONE', #8156, 1000.000000000000000 ) ;
#7195=CARTESIAN_POINT ( 'NONE',  ( 43.45299461620744808, 50.00000000000000000, 7.500000000000000000 ) ) ;
#7197=CARTESIAN_POINT ( 'NONE',  ( 43.45299461620744808, 50.00000000000000000, 7.500000000000000000 ) ) ;
#7231=DIRECTION ( 'NONE',  ( 1.000000000000000000, -0.000000000000000000, -0.000000000000000000 ) ) ;
#7236=FACE_OUTER_BOUND ( 'NONE', #5592, .T. ) ;
#7238=( LENGTH_UNIT ( ) NAMED_UNIT ( * ) SI_UNIT ( .MILLI., .METRE. ) );
#7243=DIRECTION ( 'NONE',  ( 0.000000000000000000, -0.000000000000000000, -1.000000000000000000 ) ) ;
#7269=CARTESIAN_POINT ( 'NONE',  ( 54.99999999999999289, 50.00000000000000000, 7.500000000000000000 ) ) ;
#7277=PRESENTATION_STYLE_ASSIGNMENT (( #4738 ) ) ;
#7285=ORIENTED_EDGE ( 'NONE', *, *, #3214, .F. ) ;
#7295=DIRECTION ( 'NONE',  ( 0.000000000000000000, 1.000000000000000000, 0.000000000000000000 ) ) ;
#7317=AXIS2_PLACEMENT_3D ( 'NONE', #3144, #7018, #735 ) ;
#7322=VECTOR ( 'NONE', #4032, 1000.000000000000000 ) ;
#7338=LINE ( 'NONE', #7465, #534 ) ;
#7400=AXIS2_PLACEMENT_3D ( 'NONE', #3254, #3338, #7040 ) ;
#7450=VECTOR ( 'NONE', #1591, 1000.000000000000114 ) ;
#7465=CARTESIAN_POINT ( 'NONE',  ( 75.00000000000000000, -20.00000000000000000, 7.500000000000000000 ) ) ;
#7477=EDGE_CURVE ( 'NONE', #4787, #5449, #714, .T. ) ;
#7489=ORIENTED_EDGE ( 'NONE', *, *, #3348, .T. ) ;
#7501=CYLINDRICAL_SURFACE ( 'NONE', #1468, 1.500000000000000666 ) ;
#7526=CARTESIAN_POINT ( 'NONE',  ( 75.00000000000000000, 80.00000000000000000, 7.500000000000000000 ) ) ;
#7528=ORIENTED_EDGE ( 'NONE', *, *, #1725, .T. ) ;
#7593=DIRECTION ( 'NONE',  ( 9.251858538542971828E-16, -1.000000000000000000, 0.000000000000000000 ) ) ;
#7608=ADVANCED_BREP_SHAPE_REPRESENTATION ( '', ( #1690, #2840 ), #1628 ) ;
#7652=EDGE_CURVE ( 'NONE', #5112, #5449, #8019, .T. ) ;
#7665=AXIS2_PLACEMENT_3D ( 'NONE', #2412, #6286, #3716 ) ;
#7668=DIRECTION ( 'NONE',  ( 0.000000000000000000, 0.000000000000000000, 1.000000000000000000 ) ) ;
#7669=EDGE_LOOP ( 'NONE', ( #2445, #3872, #7285, #1447 ) ) ;
#7681=LINE ( 'NONE', #7723, #646 ) ;
#7689=DIRECTION ( 'NONE',  ( -0.6099942813304201072, -0.7924058156930603447, 0.000000000000000000 ) ) ;
#7718=EDGE_CURVE ( 'NONE', #6070, #8322, #7338, .T. ) ;
#7723=CARTESIAN_POINT ( 'NONE',  ( 43.45299461620744808, 50.00000000000000000, -7.500000000000000000 ) ) ;
#7750=ORIENTED_EDGE ( 'NONE', *, *, #1659, .T. ) ;
#7806=FACE_OUTER_BOUND ( 'NONE', #3126, .T. ) ;
#7811=DIRECTION ( 'NONE',  ( 1.000000000000000000, 0.000000000000000000, 0.000000000000000000 ) ) ;
#7871=DIRECTION ( 'NONE',  ( 1.000000000000000000, 0.000000000000000000, -0.000000000000000000 ) ) ;
#7881=AXIS2_PLACEMENT_3D ( 'NONE', #5251, #912, #5970 ) ;
#7917=( NAMED_UNIT ( * ) SI_UNIT ( $, .STERADIAN. ) SOLID_ANGLE_UNIT ( ) );
#7923=ORIENTED_EDGE ( 'NONE', *, *, #4864, .T. ) ;
#7944=PLANE ( 'NONE',  #3892 ) ;
#7991=DIRECTION ( 'NONE',  ( -0.000000000000000000, 0.000000000000000000, 1.000000000000000000 ) ) ;
#8000=AXIS2_PLACEMENT_3D ( 'NONE', #393, #6087, #6717 ) ;
#8019=LINE ( 'NONE', #5352, #1623 ) ;
#8055=ORIENTED_EDGE ( 'NONE', *, *, #2178, .T. ) ;
#8120=CARTESIAN_POINT ( 'NONE',  ( 0.000000000000000000, 0.000000000000000000, 0.000000000000000000 ) ) ;
#8156=DIRECTION ( 'NONE',  ( -0.000000000000000000, -0.000000000000000000, -1.000000000000000000 ) ) ;
#8174=ORIENTED_EDGE ( 'NONE', *, *, #2393, .F. ) ;
#8176=ORIENTED_EDGE ( 'NONE', *, *, #2178, .F. ) ;
#8216=COLOUR_RGB ( '', 0.09019608, 0.27058824, 0.51372549) ;
#8279=LINE ( 'NONE', #2551, #2888 ) ;
#8303=FACE_OUTER_BOUND ( 'NONE', #6091, .T. ) ;
#8308=CARTESIAN_POINT ( 'NONE',  ( 75.00000000000000000, -20.00000000000000000, -7.500000000000000000 ) ) ;
#8319=ORIENTED_EDGE ( 'NONE', *, *, #2667, .F. ) ;
#8322=VERTEX_POINT ( 'NONE', #908 ) ;
#8323=DIRECTION ( 'NONE',  ( 0.000000000000000000, 0.000000000000000000, -1.000000000000000000 ) ) ;
ENDSEC;
END-ISO-10303-21;
